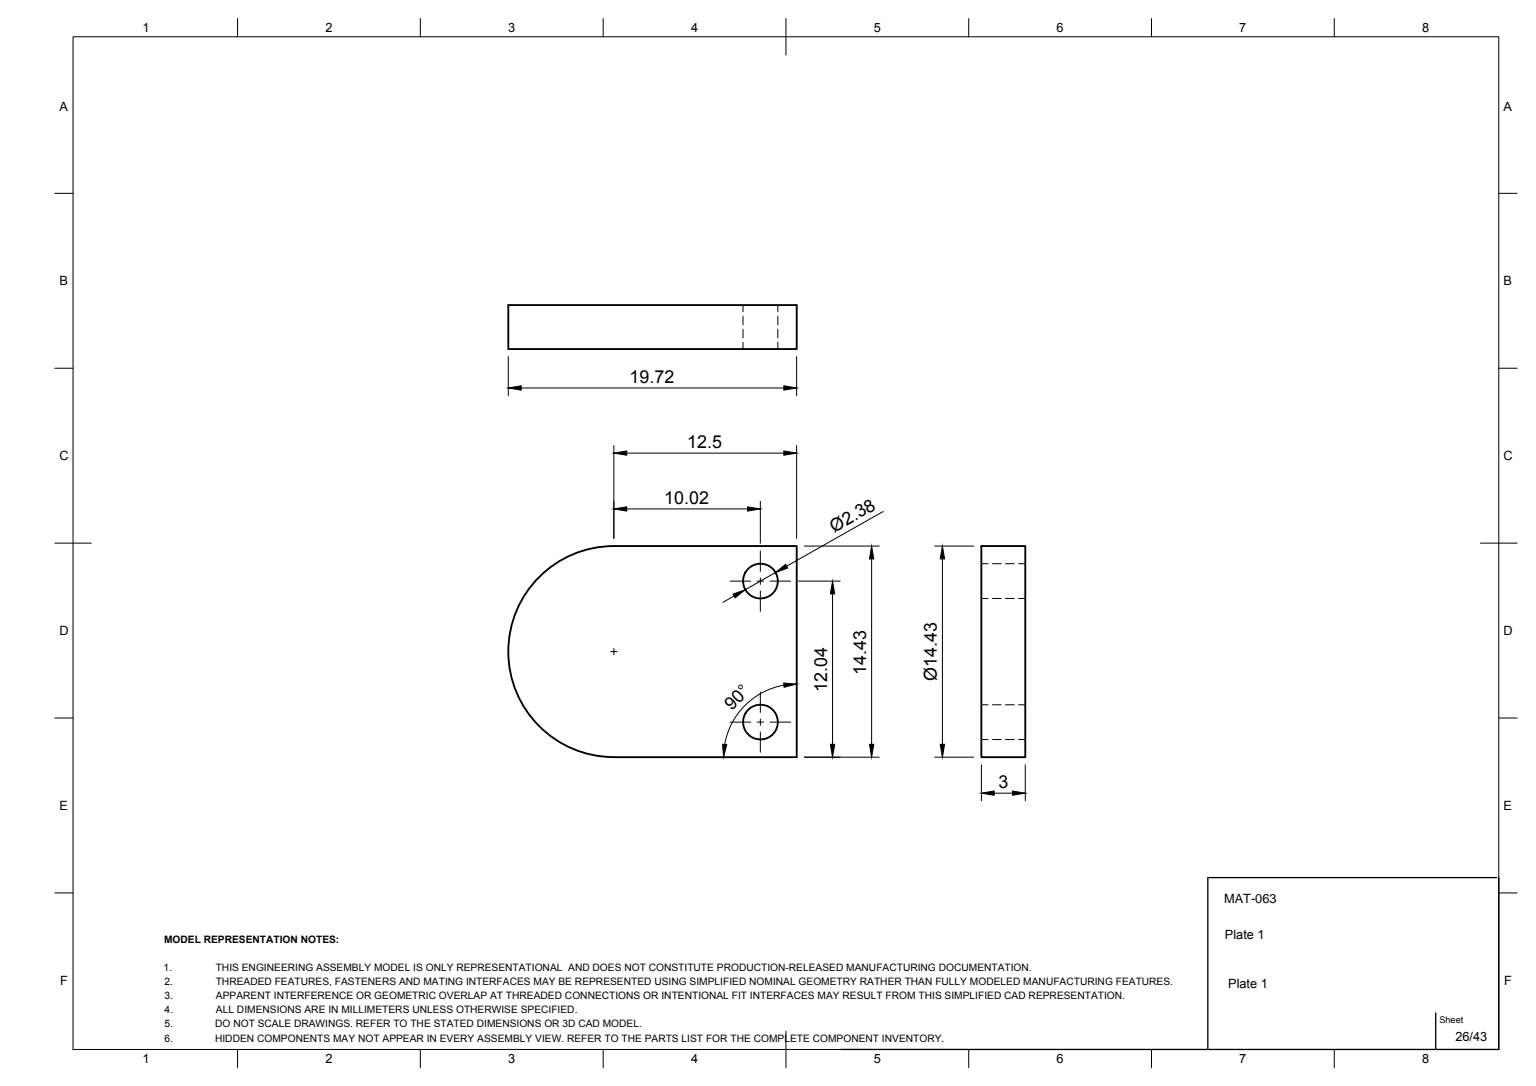
ISO-10303-21;
HEADER;
/* Generated by software containing ST-Developer
 * from STEP Tools, Inc. (www.steptools.com) 
 */

FILE_DESCRIPTION(
/* description */ (''),
/* implementation_level */ '2;1');

FILE_NAME(
/* name */ 'Plate 1.step',
/* time_stamp */ '2026-10-24T09:43:01-07:00',
/* author */ (''),
/* organization */ (''),
/* preprocessor_version */ 'ST-DEVELOPER v20.2',
/* originating_system */ 'Autodesk Translation Framework v15.15.0.0',
/* authorisation */ '');

FILE_SCHEMA (('AUTOMOTIVE_DESIGN { 1 0 10303 214 3 1 1 }'));
ENDSEC;

DATA;
#10=MECHANICAL_DESIGN_GEOMETRIC_PRESENTATION_REPRESENTATION('',(#291),#11112);
#225=SHAPE_REPRESENTATION_RELATIONSHIP('SRR','None',#11250,#258);
#258=ADVANCED_BREP_SHAPE_REPRESENTATION('',(#324),#11095);
#291=STYLED_ITEM('',(#11426),#324);
#324=MANIFOLD_SOLID_BREP('Plate 1',#6028);
#455=FACE_BOUND('',#1425,.T.);
#456=FACE_BOUND('',#1426,.T.);
#457=FACE_BOUND('',#1433,.T.);
#458=FACE_BOUND('',#1434,.T.);
#610=PLANE('',#7049);
#611=PLANE('',#7054);
#612=PLANE('',#7057);
#613=PLANE('',#7058);
#614=PLANE('',#7059);
#943=FACE_OUTER_BOUND('',#1423,.T.);
#944=FACE_OUTER_BOUND('',#1424,.T.);
#945=FACE_OUTER_BOUND('',#1427,.T.);
#946=FACE_OUTER_BOUND('',#1428,.T.);
#947=FACE_OUTER_BOUND('',#1429,.T.);
#948=FACE_OUTER_BOUND('',#1430,.T.);
#949=FACE_OUTER_BOUND('',#1431,.T.);
#950=FACE_OUTER_BOUND('',#1432,.T.);
#1423=EDGE_LOOP('',(#5113,#5114,#5115,#5116));
#1424=EDGE_LOOP('',(#5117,#5118,#5119,#5120));
#1425=EDGE_LOOP('',(#5121));
#1426=EDGE_LOOP('',(#5122));
#1427=EDGE_LOOP('',(#5123,#5124,#5125,#5126));
#1428=EDGE_LOOP('',(#5127,#5128,#5129,#5130));
#1429=EDGE_LOOP('',(#5131,#5132,#5133,#5134));
#1430=EDGE_LOOP('',(#5135,#5136,#5137,#5138));
#1431=EDGE_LOOP('',(#5139,#5140,#5141,#5142));
#1432=EDGE_LOOP('',(#5143,#5144,#5145,#5146));
#1433=EDGE_LOOP('',(#5147));
#1434=EDGE_LOOP('',(#5148));
#1798=LINE('',#10576,#2157);
#1799=LINE('',#10581,#2158);
#1800=LINE('',#10583,#2159);
#1801=LINE('',#10586,#2160);
#1802=LINE('',#10591,#2161);
#1803=LINE('',#10595,#2162);
#1804=LINE('',#10597,#2163);
#1805=LINE('',#10598,#2164);
#1806=LINE('',#10601,#2165);
#1807=LINE('',#10605,#2166);
#1808=LINE('',#10606,#2167);
#1809=LINE('',#10608,#2168);
#2157=VECTOR('',#8782,0.00118970000000007);
#2158=VECTOR('',#8787,0.01);
#2159=VECTOR('',#8788,0.01);
#2160=VECTOR('',#8791,0.01);
#2161=VECTOR('',#8796,0.00118970100000004);
#2162=VECTOR('',#8801,0.01);
#2163=VECTOR('',#8802,0.01);
#2164=VECTOR('',#8803,0.01);
#2165=VECTOR('',#8806,0.01);
#2166=VECTOR('',#8811,0.01);
#2167=VECTOR('',#8812,0.01);
#2168=VECTOR('',#8815,0.01);
#2616=CIRCLE('',#7047,0.00118970000000007);
#2617=CIRCLE('',#7048,0.00118970000000007);
#2618=CIRCLE('',#7050,0.007216878);
#2619=CIRCLE('',#7051,0.00118970100000004);
#2620=CIRCLE('',#7053,0.00118970100000004);
#2621=CIRCLE('',#7056,0.007216878);
#3050=VERTEX_POINT('',#10573);
#3051=VERTEX_POINT('',#10575);
#3052=VERTEX_POINT('',#10579);
#3053=VERTEX_POINT('',#10580);
#3054=VERTEX_POINT('',#10582);
#3055=VERTEX_POINT('',#10584);
#3056=VERTEX_POINT('',#10587);
#3057=VERTEX_POINT('',#10590);
#3058=VERTEX_POINT('',#10594);
#3059=VERTEX_POINT('',#10596);
#3060=VERTEX_POINT('',#10600);
#3061=VERTEX_POINT('',#10604);
#3760=EDGE_CURVE('',#3050,#3050,#2616,.T.);
#3761=EDGE_CURVE('',#3050,#3051,#1798,.T.);
#3762=EDGE_CURVE('',#3051,#3051,#2617,.F.);
#3763=EDGE_CURVE('',#3052,#3053,#1799,.T.);
#3764=EDGE_CURVE('',#3053,#3054,#1800,.T.);
#3765=EDGE_CURVE('',#3054,#3055,#2618,.F.);
#3766=EDGE_CURVE('',#3055,#3052,#1801,.T.);
#3767=EDGE_CURVE('',#3056,#3056,#2619,.T.);
#3768=EDGE_CURVE('',#3056,#3057,#1802,.T.);
#3769=EDGE_CURVE('',#3057,#3057,#2620,.F.);
#3770=EDGE_CURVE('',#3058,#3055,#1803,.T.);
#3771=EDGE_CURVE('',#3059,#3058,#1804,.T.);
#3772=EDGE_CURVE('',#3052,#3059,#1805,.T.);
#3773=EDGE_CURVE('',#3054,#3060,#1806,.F.);
#3774=EDGE_CURVE('',#3060,#3058,#2621,.F.);
#3775=EDGE_CURVE('',#3061,#3053,#1807,.T.);
#3776=EDGE_CURVE('',#3060,#3061,#1808,.T.);
#3777=EDGE_CURVE('',#3061,#3059,#1809,.T.);
#5113=ORIENTED_EDGE('',*,*,#3760,.F.);
#5114=ORIENTED_EDGE('',*,*,#3761,.T.);
#5115=ORIENTED_EDGE('',*,*,#3762,.F.);
#5116=ORIENTED_EDGE('',*,*,#3761,.F.);
#5117=ORIENTED_EDGE('',*,*,#3763,.T.);
#5118=ORIENTED_EDGE('',*,*,#3764,.T.);
#5119=ORIENTED_EDGE('',*,*,#3765,.T.);
#5120=ORIENTED_EDGE('',*,*,#3766,.T.);
#5121=ORIENTED_EDGE('',*,*,#3767,.T.);
#5122=ORIENTED_EDGE('',*,*,#3760,.T.);
#5123=ORIENTED_EDGE('',*,*,#3767,.F.);
#5124=ORIENTED_EDGE('',*,*,#3768,.T.);
#5125=ORIENTED_EDGE('',*,*,#3769,.F.);
#5126=ORIENTED_EDGE('',*,*,#3768,.F.);
#5127=ORIENTED_EDGE('',*,*,#3770,.F.);
#5128=ORIENTED_EDGE('',*,*,#3771,.F.);
#5129=ORIENTED_EDGE('',*,*,#3772,.F.);
#5130=ORIENTED_EDGE('',*,*,#3766,.F.);
#5131=ORIENTED_EDGE('',*,*,#3773,.T.);
#5132=ORIENTED_EDGE('',*,*,#3774,.T.);
#5133=ORIENTED_EDGE('',*,*,#3770,.T.);
#5134=ORIENTED_EDGE('',*,*,#3765,.F.);
#5135=ORIENTED_EDGE('',*,*,#3775,.F.);
#5136=ORIENTED_EDGE('',*,*,#3776,.F.);
#5137=ORIENTED_EDGE('',*,*,#3773,.F.);
#5138=ORIENTED_EDGE('',*,*,#3764,.F.);
#5139=ORIENTED_EDGE('',*,*,#3772,.T.);
#5140=ORIENTED_EDGE('',*,*,#3777,.F.);
#5141=ORIENTED_EDGE('',*,*,#3775,.T.);
#5142=ORIENTED_EDGE('',*,*,#3763,.F.);
#5143=ORIENTED_EDGE('',*,*,#3776,.T.);
#5144=ORIENTED_EDGE('',*,*,#3777,.T.);
#5145=ORIENTED_EDGE('',*,*,#3771,.T.);
#5146=ORIENTED_EDGE('',*,*,#3774,.F.);
#5147=ORIENTED_EDGE('',*,*,#3769,.T.);
#5148=ORIENTED_EDGE('',*,*,#3762,.T.);
#5607=CYLINDRICAL_SURFACE('',#7046,0.00118970000000007);
#5608=CYLINDRICAL_SURFACE('',#7052,0.00118970100000004);
#5609=CYLINDRICAL_SURFACE('',#7055,0.007216878);
#5916=ADVANCED_FACE('',(#943),#5607,.F.);
#5917=ADVANCED_FACE('',(#944,#455,#456),#610,.T.);
#5918=ADVANCED_FACE('',(#945),#5608,.F.);
#5919=ADVANCED_FACE('',(#946),#611,.F.);
#5920=ADVANCED_FACE('',(#947),#5609,.T.);
#5921=ADVANCED_FACE('',(#948),#612,.F.);
#5922=ADVANCED_FACE('',(#949),#613,.F.);
#5923=ADVANCED_FACE('',(#950,#457,#458),#614,.F.);
#6028=CLOSED_SHELL('',(#5916,#5917,#5918,#5919,#5920,#5921,#5922,#5923));
#7045=AXIS2_PLACEMENT_3D('',#10571,#8776,#8777);
#7046=AXIS2_PLACEMENT_3D('',#10572,#8778,#8779);
#7047=AXIS2_PLACEMENT_3D('',#10574,#8780,#8781);
#7048=AXIS2_PLACEMENT_3D('',#10577,#8783,#8784);
#7049=AXIS2_PLACEMENT_3D('',#10578,#8785,#8786);
#7050=AXIS2_PLACEMENT_3D('',#10585,#8789,#8790);
#7051=AXIS2_PLACEMENT_3D('',#10588,#8792,#8793);
#7052=AXIS2_PLACEMENT_3D('',#10589,#8794,#8795);
#7053=AXIS2_PLACEMENT_3D('',#10592,#8797,#8798);
#7054=AXIS2_PLACEMENT_3D('',#10593,#8799,#8800);
#7055=AXIS2_PLACEMENT_3D('',#10599,#8804,#8805);
#7056=AXIS2_PLACEMENT_3D('',#10602,#8807,#8808);
#7057=AXIS2_PLACEMENT_3D('',#10603,#8809,#8810);
#7058=AXIS2_PLACEMENT_3D('',#10607,#8813,#8814);
#7059=AXIS2_PLACEMENT_3D('',#10609,#8816,#8817);
#8776=DIRECTION('axis',(0.,0.,1.));
#8777=DIRECTION('refdir',(1.,0.,0.));
#8778=DIRECTION('center_axis',(-1.,0.,0.));
#8779=DIRECTION('ref_axis',(0.,0.,1.));
#8780=DIRECTION('center_axis',(-1.,0.,0.));
#8781=DIRECTION('ref_axis',(0.,0.,1.));
#8782=DIRECTION('',(-1.,0.,0.));
#8783=DIRECTION('center_axis',(-1.,0.,0.));
#8784=DIRECTION('ref_axis',(0.,0.,1.));
#8785=DIRECTION('center_axis',(1.,-3.89528313553954E-16,9.13571080043379E-16));
#8786=DIRECTION('ref_axis',(9.13571080043379E-16,0.,-1.));
#8787=DIRECTION('',(0.,-0.49999998104077,0.866025414730555));
#8788=DIRECTION('',(-5.68434220074081E-15,-0.866025412838334,-0.499999984318193));
#8789=DIRECTION('center_axis',(-1.,0.,0.));
#8790=DIRECTION('ref_axis',(0.,0.,1.));
#8791=DIRECTION('',(0.,0.866025392838327,0.500000018959221));
#8792=DIRECTION('center_axis',(-1.,0.,0.));
#8793=DIRECTION('ref_axis',(0.,0.,1.));
#8794=DIRECTION('center_axis',(-1.,0.,0.));
#8795=DIRECTION('ref_axis',(0.,0.,1.));
#8796=DIRECTION('',(-1.,0.,0.));
#8797=DIRECTION('center_axis',(-1.,0.,0.));
#8798=DIRECTION('ref_axis',(0.,0.,1.));
#8799=DIRECTION('center_axis',(-3.98103628970969E-15,-0.500000018959218,
0.866025392838329));
#8800=DIRECTION('ref_axis',(3.30635451599776E-31,-0.866025392838329,-0.500000018959218));
#8801=DIRECTION('',(1.,0.,0.));
#8802=DIRECTION('',(0.,-0.866025392838343,-0.500000018959194));
#8803=DIRECTION('',(-1.,0.,0.));
#8804=DIRECTION('center_axis',(-1.,0.,0.));
#8805=DIRECTION('ref_axis',(0.,-0.866025406570393,-0.499999995174586));
#8806=DIRECTION('',(1.,0.,0.));
#8807=DIRECTION('center_axis',(-1.,0.,0.));
#8808=DIRECTION('ref_axis',(0.,0.,1.));
#8809=DIRECTION('center_axis',(1.04094622668064E-14,0.499999984318195,-0.866025412838333));
#8810=DIRECTION('ref_axis',(-1.37040070007528E-32,0.866025412838333,0.499999984318195));
#8811=DIRECTION('',(1.,0.,0.));
#8812=DIRECTION('',(0.,0.866025412838317,0.499999984318223));
#8813=DIRECTION('center_axis',(6.39983061249698E-15,-0.866025414730554,
-0.499999981040772));
#8814=DIRECTION('ref_axis',(4.36001107502503E-32,0.499999981040772,-0.866025414730554));
#8815=DIRECTION('',(0.,0.499999981040781,-0.866025414730549));
#8816=DIRECTION('center_axis',(1.,7.46138741516663E-16,2.73067399561958E-16));
#8817=DIRECTION('ref_axis',(-7.46138741516663E-16,1.,-2.54006882631165E-48));
#10571=CARTESIAN_POINT('',(0.,0.,0.));
#10572=CARTESIAN_POINT('Origin',(0.493,-0.542782557,0.975695518));
#10573=CARTESIAN_POINT('',(0.493,-0.542782557,0.974505818));
#10574=CARTESIAN_POINT('Origin',(0.493,-0.542782557,0.975695518));
#10575=CARTESIAN_POINT('',(0.49,-0.542782557,0.974505818));
#10576=CARTESIAN_POINT('',(0.493,-0.542782557,0.974505818));
#10577=CARTESIAN_POINT('Origin',(0.49,-0.542782557,0.975695518));
#10578=CARTESIAN_POINT('Origin',(0.493,-0.545454380845135,0.969136388159038));
#10579=CARTESIAN_POINT('',(0.493,-0.534613544999688,0.966510345999423));
#10580=CARTESIAN_POINT('',(0.493,-0.541830423000466,0.979010345999528));
#10581=CARTESIAN_POINT('',(0.493,-0.534613544872232,0.9665103457787));
#10582=CARTESIAN_POINT('',(0.492999999985368,-0.552655740191489,0.972760346019922));
#10583=CARTESIAN_POINT('',(0.493,-0.541830423323753,0.979010345813081));
#10584=CARTESIAN_POINT('',(0.493,-0.545438862110786,0.960260346041367));
#10585=CARTESIAN_POINT('Origin',(0.493,-0.549047301,0.966510346));
#10586=CARTESIAN_POINT('',(0.493,-0.545438862219975,0.960260345872998));
#10587=CARTESIAN_POINT('',(0.493,-0.537960337,0.966153487));
#10588=CARTESIAN_POINT('Origin',(0.493,-0.537960337,0.967343188));
#10589=CARTESIAN_POINT('Origin',(0.493,-0.537960337,0.967343188));
#10590=CARTESIAN_POINT('',(0.49,-0.537960337,0.966153487));
#10591=CARTESIAN_POINT('',(0.493,-0.537960337,0.966153487));
#10592=CARTESIAN_POINT('Origin',(0.49,-0.537960337,0.967343188));
#10593=CARTESIAN_POINT('Origin',(0.4915,-0.5400262035,0.963385346000001));
#10594=CARTESIAN_POINT('',(0.490000000000001,-0.545438861975815,0.960260346119293));
#10595=CARTESIAN_POINT('',(0.490000000000002,-0.545438862,0.960260346000001));
#10596=CARTESIAN_POINT('',(0.490000000000001,-0.53461354500041,0.966510345999764));
#10597=CARTESIAN_POINT('',(0.490000000000002,-0.534613545008309,0.966510345995204));
#10598=CARTESIAN_POINT('',(0.493000000000002,-0.534613545,0.966510346000001));
#10599=CARTESIAN_POINT('Origin',(0.493,-0.549047301,0.966510346));
#10600=CARTESIAN_POINT('',(0.490000000000001,-0.552655740263515,0.972760345829652));
#10601=CARTESIAN_POINT('',(0.49000000025,-0.552655739997383,0.972760345685524));
#10602=CARTESIAN_POINT('Origin',(0.49,-0.549047301,0.966510346));
#10603=CARTESIAN_POINT('Origin',(0.4915,-0.547243082,0.975885346));
#10604=CARTESIAN_POINT('',(0.49,-0.541830423,0.979010346));
#10605=CARTESIAN_POINT('',(0.490000000000002,-0.541830423,0.979010346));
#10606=CARTESIAN_POINT('',(0.490000000000002,-0.552655740692886,0.972760346177312));
#10607=CARTESIAN_POINT('Origin',(0.4915,-0.538221983999999,0.972760345999999));
#10608=CARTESIAN_POINT('',(0.490000000000002,-0.541830422999999,0.979010346));
#10609=CARTESIAN_POINT('Origin',(0.49,-0.545454380845135,0.969136388159038));
#11056=UNCERTAINTY_MEASURE_WITH_UNIT(LENGTH_MEASURE(1.E-5),#11113,
'DISTANCE_ACCURACY_VALUE',
'Maximum model space distance between geometric entities at asserted c
onnectivities');
#11073=UNCERTAINTY_MEASURE_WITH_UNIT(LENGTH_MEASURE(1.E-5),#11113,
'DISTANCE_ACCURACY_VALUE',
'Maximum model space distance between geometric entities at asserted c
onnectivities');
#11095=(
GEOMETRIC_REPRESENTATION_CONTEXT(3)
GLOBAL_UNCERTAINTY_ASSIGNED_CONTEXT((#11056))
GLOBAL_UNIT_ASSIGNED_CONTEXT((#11113,#11114,#11115))
REPRESENTATION_CONTEXT('','3D')
);
#11112=(
GEOMETRIC_REPRESENTATION_CONTEXT(3)
GLOBAL_UNCERTAINTY_ASSIGNED_CONTEXT((#11073))
GLOBAL_UNIT_ASSIGNED_CONTEXT((#11113,#11114,#11115))
REPRESENTATION_CONTEXT('','3D')
);
#11113=(
LENGTH_UNIT()
NAMED_UNIT(*)
SI_UNIT($,.METRE.)
);
#11114=(
NAMED_UNIT(*)
PLANE_ANGLE_UNIT()
SI_UNIT($,.RADIAN.)
);
#11115=(
NAMED_UNIT(*)
SI_UNIT($,.STERADIAN.)
SOLID_ANGLE_UNIT()
);
#11137=SHAPE_DEFINITION_REPRESENTATION(#11182,#11250);
#11182=PRODUCT_DEFINITION_SHAPE('',$,#11289);
#11250=SHAPE_REPRESENTATION('',(#7045),#11095);
#11267=PRODUCT_DEFINITION_CONTEXT('part definition',#11383,'design');
#11289=PRODUCT_DEFINITION('Plate 1','Plate 1',#11327,#11267);
#11327=PRODUCT_DEFINITION_FORMATION('',$,#11406);
#11383=APPLICATION_CONTEXT(
'Core Data for Automotive Mechanical Design Process');
#11384=PRODUCT_CONTEXT('part definition',#11383,'mechanical');
#11406=PRODUCT('Plate 1','Plate 1','all_plates__ DE     1939',(#11384));
#11426=PRESENTATION_STYLE_ASSIGNMENT((#11430));
#11430=SURFACE_STYLE_USAGE(.BOTH.,#11434);
#11434=SURFACE_SIDE_STYLE('',(#11438));
#11438=SURFACE_STYLE_FILL_AREA(#11442);
#11442=FILL_AREA_STYLE('Opaque(202,209,238)',(#11446));
#11446=FILL_AREA_STYLE_COLOUR('Opaque(202,209,238)',#11450);
#11450=COLOUR_RGB('Opaque(202,209,238)',0.792156862745098,0.819607843137255,
0.933333333333333);
ENDSEC;
END-ISO-10303-21;
